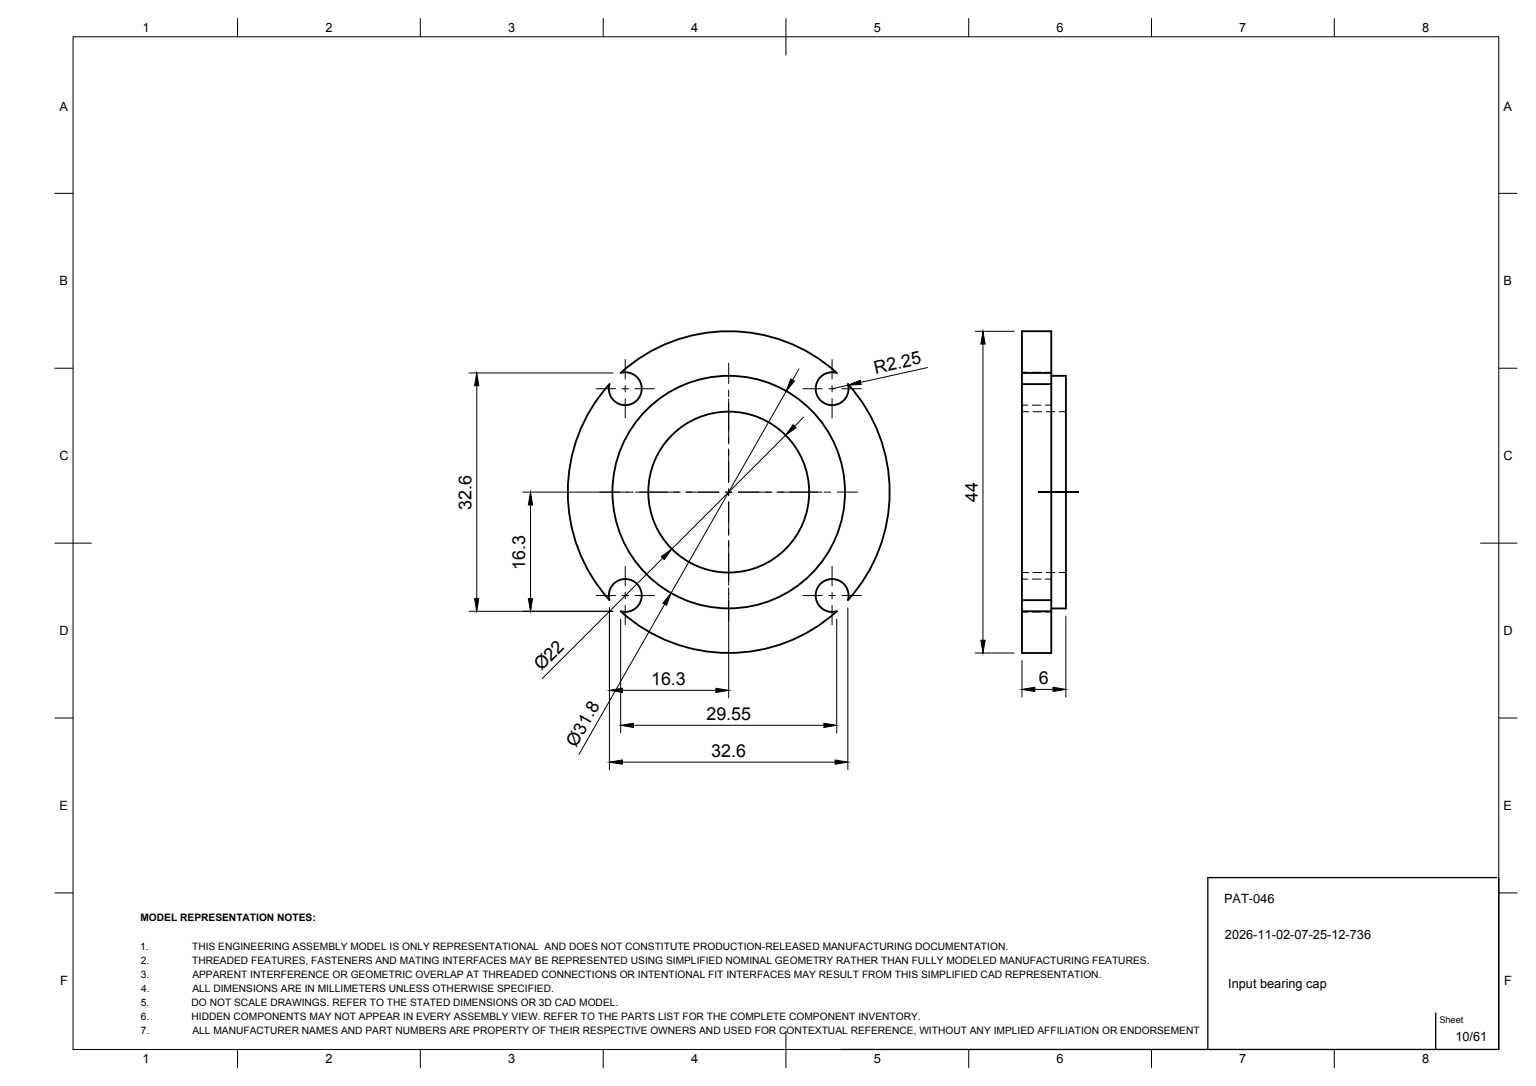
ISO-10303-21;
HEADER;
/* Generated by software containing ST-Developer
 * from STEP Tools, Inc. (www.steptools.com) 
 */

FILE_DESCRIPTION(
/* description */ ('Gear mesh backlash fixture'),
/* implementation_level */ '2;1');

FILE_NAME(
/* name */ 'Input bearing cap.step',
/* time_stamp */ '2026-10-28T03:26:00-07:00',
/* author */ (''),
/* organization */ (''),
/* preprocessor_version */ 'ST-DEVELOPER v20.2',
/* originating_system */ 'Autodesk Translation Framework v15.17.0.0',
/* authorisation */ '');

FILE_SCHEMA (('AUTOMOTIVE_DESIGN { 1 0 10303 214 3 1 1 }'));
ENDSEC;

DATA;
#10=MECHANICAL_DESIGN_GEOMETRIC_PRESENTATION_REPRESENTATION('',(#1021),#57900);
#921=SHAPE_REPRESENTATION_RELATIONSHIP('SRR','None',#58116,#971);
#971=ADVANCED_BREP_SHAPE_REPRESENTATION('',(#1086),#57849);
#1021=STYLED_ITEM('',(#58465),#1086);
#1086=MANIFOLD_SOLID_BREP('Body1',#13581);
#1187=FACE_BOUND('',#2571,.T.);
#1188=FACE_BOUND('',#2578,.T.);
#1189=FACE_BOUND('',#2581,.T.);
#1362=PLANE('',#14346);
#1363=PLANE('',#14362);
#1364=PLANE('',#14366);
#1757=FACE_OUTER_BOUND('',#2566,.T.);
#1758=FACE_OUTER_BOUND('',#2567,.T.);
#1759=FACE_OUTER_BOUND('',#2568,.T.);
#1760=FACE_OUTER_BOUND('',#2569,.T.);
#1761=FACE_OUTER_BOUND('',#2570,.T.);
#1762=FACE_OUTER_BOUND('',#2572,.T.);
#1763=FACE_OUTER_BOUND('',#2573,.T.);
#1764=FACE_OUTER_BOUND('',#2574,.T.);
#1765=FACE_OUTER_BOUND('',#2575,.T.);
#1766=FACE_OUTER_BOUND('',#2576,.T.);
#1767=FACE_OUTER_BOUND('',#2577,.T.);
#1768=FACE_OUTER_BOUND('',#2579,.T.);
#1769=FACE_OUTER_BOUND('',#2580,.T.);
#2566=EDGE_LOOP('',(#9165,#9166,#9167,#9168));
#2567=EDGE_LOOP('',(#9169,#9170,#9171,#9172));
#2568=EDGE_LOOP('',(#9173,#9174,#9175,#9176));
#2569=EDGE_LOOP('',(#9177,#9178,#9179,#9180));
#2570=EDGE_LOOP('',(#9181,#9182,#9183,#9184,#9185,#9186,#9187,#9188));
#2571=EDGE_LOOP('',(#9189));
#2572=EDGE_LOOP('',(#9190,#9191,#9192,#9193));
#2573=EDGE_LOOP('',(#9194,#9195,#9196,#9197));
#2574=EDGE_LOOP('',(#9198,#9199,#9200,#9201));
#2575=EDGE_LOOP('',(#9202,#9203,#9204,#9205));
#2576=EDGE_LOOP('',(#9206,#9207,#9208,#9209));
#2577=EDGE_LOOP('',(#9210));
#2578=EDGE_LOOP('',(#9211));
#2579=EDGE_LOOP('',(#9212,#9213,#9214,#9215));
#2580=EDGE_LOOP('',(#9216,#9217,#9218,#9219,#9220,#9221,#9222,#9223));
#2581=EDGE_LOOP('',(#9224));
#3482=LINE('',#19614,#4371);
#3483=LINE('',#19618,#4372);
#3484=LINE('',#19623,#4373);
#3485=LINE('',#19627,#4374);
#3486=LINE('',#19632,#4375);
#3487=LINE('',#19636,#4376);
#3488=LINE('',#19641,#4377);
#3489=LINE('',#19645,#4378);
#3490=LINE('',#19664,#4379);
#3491=LINE('',#19672,#4380);
#4371=VECTOR('',#15929,1.);
#4372=VECTOR('',#15932,1.);
#4373=VECTOR('',#15937,1.);
#4374=VECTOR('',#15940,1.);
#4375=VECTOR('',#15945,1.);
#4376=VECTOR('',#15948,1.);
#4377=VECTOR('',#15953,1.);
#4378=VECTOR('',#15956,1.);
#4379=VECTOR('',#15989,1.59);
#4380=VECTOR('',#16000,1.1);
#5257=CIRCLE('',#14335,0.225);
#5258=CIRCLE('',#14336,0.225);
#5259=CIRCLE('',#14338,0.225);
#5260=CIRCLE('',#14339,0.225);
#5261=CIRCLE('',#14341,0.225);
#5262=CIRCLE('',#14342,0.225);
#5263=CIRCLE('',#14344,0.225);
#5264=CIRCLE('',#14345,0.225);
#5265=CIRCLE('',#14347,2.2);
#5266=CIRCLE('',#14348,2.2);
#5267=CIRCLE('',#14349,2.2);
#5268=CIRCLE('',#14350,2.2);
#5269=CIRCLE('',#14351,1.59);
#5270=CIRCLE('',#14353,2.2);
#5271=CIRCLE('',#14355,2.2);
#5272=CIRCLE('',#14357,2.2);
#5273=CIRCLE('',#14359,2.2);
#5274=CIRCLE('',#14361,1.59);
#5275=CIRCLE('',#14363,1.1);
#5276=CIRCLE('',#14365,1.1);
#5877=VERTEX_POINT('',#19612);
#5878=VERTEX_POINT('',#19613);
#5879=VERTEX_POINT('',#19615);
#5880=VERTEX_POINT('',#19617);
#5881=VERTEX_POINT('',#19621);
#5882=VERTEX_POINT('',#19622);
#5883=VERTEX_POINT('',#19624);
#5884=VERTEX_POINT('',#19626);
#5885=VERTEX_POINT('',#19630);
#5886=VERTEX_POINT('',#19631);
#5887=VERTEX_POINT('',#19633);
#5888=VERTEX_POINT('',#19635);
#5889=VERTEX_POINT('',#19639);
#5890=VERTEX_POINT('',#19640);
#5891=VERTEX_POINT('',#19642);
#5892=VERTEX_POINT('',#19644);
#5893=VERTEX_POINT('',#19652);
#5894=VERTEX_POINT('',#19663);
#5895=VERTEX_POINT('',#19667);
#5896=VERTEX_POINT('',#19670);
#7169=EDGE_CURVE('',#5877,#5878,#3482,.T.);
#7170=EDGE_CURVE('',#5879,#5877,#5257,.T.);
#7171=EDGE_CURVE('',#5880,#5879,#3483,.T.);
#7172=EDGE_CURVE('',#5878,#5880,#5258,.T.);
#7173=EDGE_CURVE('',#5881,#5882,#3484,.T.);
#7174=EDGE_CURVE('',#5883,#5881,#5259,.T.);
#7175=EDGE_CURVE('',#5884,#5883,#3485,.T.);
#7176=EDGE_CURVE('',#5882,#5884,#5260,.T.);
#7177=EDGE_CURVE('',#5885,#5886,#3486,.T.);
#7178=EDGE_CURVE('',#5887,#5885,#5261,.T.);
#7179=EDGE_CURVE('',#5888,#5887,#3487,.T.);
#7180=EDGE_CURVE('',#5886,#5888,#5262,.T.);
#7181=EDGE_CURVE('',#5889,#5890,#3488,.T.);
#7182=EDGE_CURVE('',#5891,#5889,#5263,.T.);
#7183=EDGE_CURVE('',#5892,#5891,#3489,.T.);
#7184=EDGE_CURVE('',#5890,#5892,#5264,.T.);
#7185=EDGE_CURVE('',#5883,#5877,#5265,.T.);
#7186=EDGE_CURVE('',#5887,#5881,#5266,.T.);
#7187=EDGE_CURVE('',#5891,#5885,#5267,.T.);
#7188=EDGE_CURVE('',#5879,#5889,#5268,.T.);
#7189=EDGE_CURVE('',#5893,#5893,#5269,.T.);
#7190=EDGE_CURVE('',#5892,#5886,#5270,.T.);
#7191=EDGE_CURVE('',#5888,#5882,#5271,.T.);
#7192=EDGE_CURVE('',#5884,#5878,#5272,.T.);
#7193=EDGE_CURVE('',#5880,#5890,#5273,.T.);
#7194=EDGE_CURVE('',#5893,#5894,#3490,.T.);
#7195=EDGE_CURVE('',#5894,#5894,#5274,.T.);
#7196=EDGE_CURVE('',#5895,#5895,#5275,.T.);
#7197=EDGE_CURVE('',#5896,#5896,#5276,.T.);
#7198=EDGE_CURVE('',#5896,#5895,#3491,.T.);
#9165=ORIENTED_EDGE('',*,*,#7169,.F.);
#9166=ORIENTED_EDGE('',*,*,#7170,.F.);
#9167=ORIENTED_EDGE('',*,*,#7171,.F.);
#9168=ORIENTED_EDGE('',*,*,#7172,.F.);
#9169=ORIENTED_EDGE('',*,*,#7173,.F.);
#9170=ORIENTED_EDGE('',*,*,#7174,.F.);
#9171=ORIENTED_EDGE('',*,*,#7175,.F.);
#9172=ORIENTED_EDGE('',*,*,#7176,.F.);
#9173=ORIENTED_EDGE('',*,*,#7177,.F.);
#9174=ORIENTED_EDGE('',*,*,#7178,.F.);
#9175=ORIENTED_EDGE('',*,*,#7179,.F.);
#9176=ORIENTED_EDGE('',*,*,#7180,.F.);
#9177=ORIENTED_EDGE('',*,*,#7181,.F.);
#9178=ORIENTED_EDGE('',*,*,#7182,.F.);
#9179=ORIENTED_EDGE('',*,*,#7183,.F.);
#9180=ORIENTED_EDGE('',*,*,#7184,.F.);
#9181=ORIENTED_EDGE('',*,*,#7170,.T.);
#9182=ORIENTED_EDGE('',*,*,#7185,.F.);
#9183=ORIENTED_EDGE('',*,*,#7174,.T.);
#9184=ORIENTED_EDGE('',*,*,#7186,.F.);
#9185=ORIENTED_EDGE('',*,*,#7178,.T.);
#9186=ORIENTED_EDGE('',*,*,#7187,.F.);
#9187=ORIENTED_EDGE('',*,*,#7182,.T.);
#9188=ORIENTED_EDGE('',*,*,#7188,.F.);
#9189=ORIENTED_EDGE('',*,*,#7189,.T.);
#9190=ORIENTED_EDGE('',*,*,#7177,.T.);
#9191=ORIENTED_EDGE('',*,*,#7190,.F.);
#9192=ORIENTED_EDGE('',*,*,#7183,.T.);
#9193=ORIENTED_EDGE('',*,*,#7187,.T.);
#9194=ORIENTED_EDGE('',*,*,#7173,.T.);
#9195=ORIENTED_EDGE('',*,*,#7191,.F.);
#9196=ORIENTED_EDGE('',*,*,#7179,.T.);
#9197=ORIENTED_EDGE('',*,*,#7186,.T.);
#9198=ORIENTED_EDGE('',*,*,#7169,.T.);
#9199=ORIENTED_EDGE('',*,*,#7192,.F.);
#9200=ORIENTED_EDGE('',*,*,#7175,.T.);
#9201=ORIENTED_EDGE('',*,*,#7185,.T.);
#9202=ORIENTED_EDGE('',*,*,#7171,.T.);
#9203=ORIENTED_EDGE('',*,*,#7188,.T.);
#9204=ORIENTED_EDGE('',*,*,#7181,.T.);
#9205=ORIENTED_EDGE('',*,*,#7193,.F.);
#9206=ORIENTED_EDGE('',*,*,#7189,.F.);
#9207=ORIENTED_EDGE('',*,*,#7194,.T.);
#9208=ORIENTED_EDGE('',*,*,#7195,.T.);
#9209=ORIENTED_EDGE('',*,*,#7194,.F.);
#9210=ORIENTED_EDGE('',*,*,#7195,.F.);
#9211=ORIENTED_EDGE('',*,*,#7196,.F.);
#9212=ORIENTED_EDGE('',*,*,#7197,.F.);
#9213=ORIENTED_EDGE('',*,*,#7198,.T.);
#9214=ORIENTED_EDGE('',*,*,#7196,.T.);
#9215=ORIENTED_EDGE('',*,*,#7198,.F.);
#9216=ORIENTED_EDGE('',*,*,#7172,.T.);
#9217=ORIENTED_EDGE('',*,*,#7193,.T.);
#9218=ORIENTED_EDGE('',*,*,#7184,.T.);
#9219=ORIENTED_EDGE('',*,*,#7190,.T.);
#9220=ORIENTED_EDGE('',*,*,#7180,.T.);
#9221=ORIENTED_EDGE('',*,*,#7191,.T.);
#9222=ORIENTED_EDGE('',*,*,#7176,.T.);
#9223=ORIENTED_EDGE('',*,*,#7192,.T.);
#9224=ORIENTED_EDGE('',*,*,#7197,.T.);
#12616=CYLINDRICAL_SURFACE('',#14334,0.225);
#12617=CYLINDRICAL_SURFACE('',#14337,0.225);
#12618=CYLINDRICAL_SURFACE('',#14340,0.225);
#12619=CYLINDRICAL_SURFACE('',#14343,0.225);
#12620=CYLINDRICAL_SURFACE('',#14352,2.2);
#12621=CYLINDRICAL_SURFACE('',#14354,2.2);
#12622=CYLINDRICAL_SURFACE('',#14356,2.2);
#12623=CYLINDRICAL_SURFACE('',#14358,2.2);
#12624=CYLINDRICAL_SURFACE('',#14360,1.59);
#12625=CYLINDRICAL_SURFACE('',#14364,1.1);
#12874=ADVANCED_FACE('',(#1757),#12616,.F.);
#12875=ADVANCED_FACE('',(#1758),#12617,.F.);
#12876=ADVANCED_FACE('',(#1759),#12618,.F.);
#12877=ADVANCED_FACE('',(#1760),#12619,.F.);
#12878=ADVANCED_FACE('',(#1761,#1187),#1362,.F.);
#12879=ADVANCED_FACE('',(#1762),#12620,.T.);
#12880=ADVANCED_FACE('',(#1763),#12621,.T.);
#12881=ADVANCED_FACE('',(#1764),#12622,.T.);
#12882=ADVANCED_FACE('',(#1765),#12623,.T.);
#12883=ADVANCED_FACE('',(#1766),#12624,.T.);
#12884=ADVANCED_FACE('',(#1767,#1188),#1363,.F.);
#12885=ADVANCED_FACE('',(#1768),#12625,.F.);
#12886=ADVANCED_FACE('',(#1769,#1189),#1364,.T.);
#13581=CLOSED_SHELL('',(#12874,#12875,#12876,#12877,#12878,#12879,#12880,
#12881,#12882,#12883,#12884,#12885,#12886));
#14333=AXIS2_PLACEMENT_3D('',#19610,#15925,#15926);
#14334=AXIS2_PLACEMENT_3D('',#19611,#15927,#15928);
#14335=AXIS2_PLACEMENT_3D('',#19616,#15930,#15931);
#14336=AXIS2_PLACEMENT_3D('',#19619,#15933,#15934);
#14337=AXIS2_PLACEMENT_3D('',#19620,#15935,#15936);
#14338=AXIS2_PLACEMENT_3D('',#19625,#15938,#15939);
#14339=AXIS2_PLACEMENT_3D('',#19628,#15941,#15942);
#14340=AXIS2_PLACEMENT_3D('',#19629,#15943,#15944);
#14341=AXIS2_PLACEMENT_3D('',#19634,#15946,#15947);
#14342=AXIS2_PLACEMENT_3D('',#19637,#15949,#15950);
#14343=AXIS2_PLACEMENT_3D('',#19638,#15951,#15952);
#14344=AXIS2_PLACEMENT_3D('',#19643,#15954,#15955);
#14345=AXIS2_PLACEMENT_3D('',#19646,#15957,#15958);
#14346=AXIS2_PLACEMENT_3D('',#19647,#15959,#15960);
#14347=AXIS2_PLACEMENT_3D('',#19648,#15961,#15962);
#14348=AXIS2_PLACEMENT_3D('',#19649,#15963,#15964);
#14349=AXIS2_PLACEMENT_3D('',#19650,#15965,#15966);
#14350=AXIS2_PLACEMENT_3D('',#19651,#15967,#15968);
#14351=AXIS2_PLACEMENT_3D('',#19653,#15969,#15970);
#14352=AXIS2_PLACEMENT_3D('',#19654,#15971,#15972);
#14353=AXIS2_PLACEMENT_3D('',#19655,#15973,#15974);
#14354=AXIS2_PLACEMENT_3D('',#19656,#15975,#15976);
#14355=AXIS2_PLACEMENT_3D('',#19657,#15977,#15978);
#14356=AXIS2_PLACEMENT_3D('',#19658,#15979,#15980);
#14357=AXIS2_PLACEMENT_3D('',#19659,#15981,#15982);
#14358=AXIS2_PLACEMENT_3D('',#19660,#15983,#15984);
#14359=AXIS2_PLACEMENT_3D('',#19661,#15985,#15986);
#14360=AXIS2_PLACEMENT_3D('',#19662,#15987,#15988);
#14361=AXIS2_PLACEMENT_3D('',#19665,#15990,#15991);
#14362=AXIS2_PLACEMENT_3D('',#19666,#15992,#15993);
#14363=AXIS2_PLACEMENT_3D('',#19668,#15994,#15995);
#14364=AXIS2_PLACEMENT_3D('',#19669,#15996,#15997);
#14365=AXIS2_PLACEMENT_3D('',#19671,#15998,#15999);
#14366=AXIS2_PLACEMENT_3D('',#19673,#16001,#16002);
#15925=DIRECTION('axis',(0.,0.,1.));
#15926=DIRECTION('refdir',(1.,0.,0.));
#15927=DIRECTION('center_axis',(0.,0.,1.));
#15928=DIRECTION('ref_axis',(0.707106781186547,0.707106781186548,0.));
#15929=DIRECTION('',(0.,0.,1.));
#15930=DIRECTION('center_axis',(0.,0.,1.));
#15931=DIRECTION('ref_axis',(1.,0.,0.));
#15932=DIRECTION('',(0.,0.,-1.));
#15933=DIRECTION('center_axis',(0.,0.,-1.));
#15934=DIRECTION('ref_axis',(1.,0.,0.));
#15935=DIRECTION('center_axis',(0.,0.,1.));
#15936=DIRECTION('ref_axis',(0.707106781186548,-0.707106781186547,0.));
#15937=DIRECTION('',(0.,0.,1.));
#15938=DIRECTION('center_axis',(0.,0.,1.));
#15939=DIRECTION('ref_axis',(1.,0.,0.));
#15940=DIRECTION('',(0.,0.,-1.));
#15941=DIRECTION('center_axis',(0.,0.,-1.));
#15942=DIRECTION('ref_axis',(1.,0.,0.));
#15943=DIRECTION('center_axis',(0.,0.,1.));
#15944=DIRECTION('ref_axis',(-0.707106781186547,-0.707106781186548,0.));
#15945=DIRECTION('',(0.,0.,1.));
#15946=DIRECTION('center_axis',(0.,0.,1.));
#15947=DIRECTION('ref_axis',(1.,0.,0.));
#15948=DIRECTION('',(0.,0.,-1.));
#15949=DIRECTION('center_axis',(0.,0.,-1.));
#15950=DIRECTION('ref_axis',(1.,0.,0.));
#15951=DIRECTION('center_axis',(0.,0.,1.));
#15952=DIRECTION('ref_axis',(-0.707106781186548,0.707106781186547,0.));
#15953=DIRECTION('',(0.,0.,1.));
#15954=DIRECTION('center_axis',(0.,0.,1.));
#15955=DIRECTION('ref_axis',(1.,0.,0.));
#15956=DIRECTION('',(0.,0.,-1.));
#15957=DIRECTION('center_axis',(0.,0.,-1.));
#15958=DIRECTION('ref_axis',(1.,0.,0.));
#15959=DIRECTION('center_axis',(0.,0.,1.));
#15960=DIRECTION('ref_axis',(1.,0.,0.));
#15961=DIRECTION('center_axis',(0.,0.,1.));
#15962=DIRECTION('ref_axis',(1.,0.,0.));
#15963=DIRECTION('center_axis',(0.,0.,1.));
#15964=DIRECTION('ref_axis',(1.,0.,0.));
#15965=DIRECTION('center_axis',(0.,0.,1.));
#15966=DIRECTION('ref_axis',(1.,0.,0.));
#15967=DIRECTION('center_axis',(0.,0.,1.));
#15968=DIRECTION('ref_axis',(1.,0.,0.));
#15969=DIRECTION('center_axis',(0.,0.,1.));
#15970=DIRECTION('ref_axis',(1.,0.,0.));
#15971=DIRECTION('center_axis',(0.,0.,1.));
#15972=DIRECTION('ref_axis',(1.,0.,0.));
#15973=DIRECTION('center_axis',(0.,0.,1.));
#15974=DIRECTION('ref_axis',(1.,0.,0.));
#15975=DIRECTION('center_axis',(0.,0.,1.));
#15976=DIRECTION('ref_axis',(1.,0.,0.));
#15977=DIRECTION('center_axis',(0.,0.,1.));
#15978=DIRECTION('ref_axis',(1.,0.,0.));
#15979=DIRECTION('center_axis',(0.,0.,1.));
#15980=DIRECTION('ref_axis',(-1.,-1.22464679914735E-16,0.));
#15981=DIRECTION('center_axis',(0.,0.,1.));
#15982=DIRECTION('ref_axis',(1.,0.,0.));
#15983=DIRECTION('center_axis',(0.,0.,1.));
#15984=DIRECTION('ref_axis',(1.,0.,0.));
#15985=DIRECTION('center_axis',(0.,0.,1.));
#15986=DIRECTION('ref_axis',(1.,0.,0.));
#15987=DIRECTION('center_axis',(0.,0.,1.));
#15988=DIRECTION('ref_axis',(1.,0.,0.));
#15989=DIRECTION('',(0.,0.,-1.));
#15990=DIRECTION('center_axis',(0.,0.,1.));
#15991=DIRECTION('ref_axis',(1.,0.,0.));
#15992=DIRECTION('center_axis',(0.,0.,1.));
#15993=DIRECTION('ref_axis',(1.,0.,0.));
#15994=DIRECTION('center_axis',(0.,0.,-1.));
#15995=DIRECTION('ref_axis',(1.,0.,0.));
#15996=DIRECTION('center_axis',(0.,0.,1.));
#15997=DIRECTION('ref_axis',(1.,0.,0.));
#15998=DIRECTION('center_axis',(0.,0.,-1.));
#15999=DIRECTION('ref_axis',(1.,0.,0.));
#16000=DIRECTION('',(0.,0.,-1.));
#16001=DIRECTION('center_axis',(0.,0.,1.));
#16002=DIRECTION('ref_axis',(1.,0.,0.));
#19610=CARTESIAN_POINT('',(0.,0.,0.));
#19611=CARTESIAN_POINT('Origin',(-1.4142135623731,-1.41421356237309,9.1));
#19612=CARTESIAN_POINT('',(-1.6301780125076,-1.47733531993816,9.2));
#19613=CARTESIAN_POINT('',(-1.6301780125076,-1.47733531993816,9.6));
#19614=CARTESIAN_POINT('',(-1.6301780125076,-1.47733531993816,9.1));
#19615=CARTESIAN_POINT('',(-1.47733531993816,-1.6301780125076,9.2));
#19616=CARTESIAN_POINT('Origin',(-1.4142135623731,-1.41421356237309,9.2));
#19617=CARTESIAN_POINT('',(-1.47733531993816,-1.6301780125076,9.6));
#19618=CARTESIAN_POINT('',(-1.47733531993816,-1.6301780125076,9.1));
#19619=CARTESIAN_POINT('Origin',(-1.4142135623731,-1.41421356237309,9.6));
#19620=CARTESIAN_POINT('Origin',(-1.41421356237309,1.4142135623731,9.1));
#19621=CARTESIAN_POINT('',(-1.47733531993816,1.6301780125076,9.2));
#19622=CARTESIAN_POINT('',(-1.47733531993816,1.6301780125076,9.6));
#19623=CARTESIAN_POINT('',(-1.47733531993816,1.6301780125076,9.1));
#19624=CARTESIAN_POINT('',(-1.6301780125076,1.47733531993816,9.2));
#19625=CARTESIAN_POINT('Origin',(-1.41421356237309,1.4142135623731,9.2));
#19626=CARTESIAN_POINT('',(-1.6301780125076,1.47733531993816,9.6));
#19627=CARTESIAN_POINT('',(-1.6301780125076,1.47733531993816,9.1));
#19628=CARTESIAN_POINT('Origin',(-1.41421356237309,1.4142135623731,9.6));
#19629=CARTESIAN_POINT('Origin',(1.4142135623731,1.41421356237309,9.1));
#19630=CARTESIAN_POINT('',(1.6301780125076,1.47733531993816,9.2));
#19631=CARTESIAN_POINT('',(1.6301780125076,1.47733531993816,9.6));
#19632=CARTESIAN_POINT('',(1.6301780125076,1.47733531993816,9.1));
#19633=CARTESIAN_POINT('',(1.47733531993816,1.6301780125076,9.2));
#19634=CARTESIAN_POINT('Origin',(1.4142135623731,1.41421356237309,9.2));
#19635=CARTESIAN_POINT('',(1.47733531993816,1.6301780125076,9.6));
#19636=CARTESIAN_POINT('',(1.47733531993816,1.6301780125076,9.1));
#19637=CARTESIAN_POINT('Origin',(1.4142135623731,1.41421356237309,9.6));
#19638=CARTESIAN_POINT('Origin',(1.41421356237309,-1.4142135623731,9.1));
#19639=CARTESIAN_POINT('',(1.47733531993816,-1.6301780125076,9.2));
#19640=CARTESIAN_POINT('',(1.47733531993816,-1.6301780125076,9.6));
#19641=CARTESIAN_POINT('',(1.47733531993816,-1.6301780125076,9.1));
#19642=CARTESIAN_POINT('',(1.6301780125076,-1.47733531993816,9.2));
#19643=CARTESIAN_POINT('Origin',(1.41421356237309,-1.4142135623731,9.2));
#19644=CARTESIAN_POINT('',(1.6301780125076,-1.47733531993816,9.6));
#19645=CARTESIAN_POINT('',(1.6301780125076,-1.47733531993816,9.1));
#19646=CARTESIAN_POINT('Origin',(1.41421356237309,-1.4142135623731,9.6));
#19647=CARTESIAN_POINT('Origin',(0.,0.,9.2));
#19648=CARTESIAN_POINT('Origin',(0.,0.,9.2));
#19649=CARTESIAN_POINT('Origin',(0.,0.,9.2));
#19650=CARTESIAN_POINT('Origin',(0.,0.,9.2));
#19651=CARTESIAN_POINT('Origin',(0.,0.,9.2));
#19652=CARTESIAN_POINT('',(-1.59,-1.94718841064429E-16,9.2));
#19653=CARTESIAN_POINT('Origin',(0.,0.,9.2));
#19654=CARTESIAN_POINT('Origin',(0.,0.,9.2));
#19655=CARTESIAN_POINT('Origin',(0.,0.,9.6));
#19656=CARTESIAN_POINT('Origin',(0.,0.,9.2));
#19657=CARTESIAN_POINT('Origin',(0.,0.,9.6));
#19658=CARTESIAN_POINT('Origin',(0.,0.,9.2));
#19659=CARTESIAN_POINT('Origin',(0.,0.,9.6));
#19660=CARTESIAN_POINT('Origin',(0.,0.,9.2));
#19661=CARTESIAN_POINT('Origin',(0.,0.,9.6));
#19662=CARTESIAN_POINT('Origin',(0.,0.,9.));
#19663=CARTESIAN_POINT('',(-1.59,-1.94718841064429E-16,9.));
#19664=CARTESIAN_POINT('',(-1.59,-1.94718841064429E-16,9.));
#19665=CARTESIAN_POINT('Origin',(0.,0.,9.));
#19666=CARTESIAN_POINT('Origin',(0.,0.,9.));
#19667=CARTESIAN_POINT('',(-1.1,-1.34711147906209E-16,9.));
#19668=CARTESIAN_POINT('Origin',(0.,0.,9.));
#19669=CARTESIAN_POINT('Origin',(0.,0.,9.2));
#19670=CARTESIAN_POINT('',(-1.1,-1.34711147906209E-16,9.6));
#19671=CARTESIAN_POINT('Origin',(0.,0.,9.6));
#19672=CARTESIAN_POINT('',(-1.1,-1.34711147906209E-16,9.2));
#19673=CARTESIAN_POINT('Origin',(0.,0.,9.6));
#57790=UNCERTAINTY_MEASURE_WITH_UNIT(LENGTH_MEASURE(0.001),#57901,
'DISTANCE_ACCURACY_VALUE',
'Maximum model space distance between geometric entities at asserted c
onnectivities');
#57841=UNCERTAINTY_MEASURE_WITH_UNIT(LENGTH_MEASURE(0.001),#57901,
'DISTANCE_ACCURACY_VALUE',
'Maximum model space distance between geometric entities at asserted c
onnectivities');
#57849=(
GEOMETRIC_REPRESENTATION_CONTEXT(3)
GLOBAL_UNCERTAINTY_ASSIGNED_CONTEXT((#57790))
GLOBAL_UNIT_ASSIGNED_CONTEXT((#57901,#57903,#57904))
REPRESENTATION_CONTEXT('','3D')
);
#57900=(
GEOMETRIC_REPRESENTATION_CONTEXT(3)
GLOBAL_UNCERTAINTY_ASSIGNED_CONTEXT((#57841))
GLOBAL_UNIT_ASSIGNED_CONTEXT((#57901,#57903,#57904))
REPRESENTATION_CONTEXT('','3D')
);
#57901=(
LENGTH_UNIT()
NAMED_UNIT(*)
SI_UNIT(.CENTI.,.METRE.)
);
#57903=(
NAMED_UNIT(*)
PLANE_ANGLE_UNIT()
SI_UNIT($,.RADIAN.)
);
#57904=(
NAMED_UNIT(*)
SI_UNIT($,.STERADIAN.)
SOLID_ANGLE_UNIT()
);
#57912=SHAPE_DEFINITION_REPRESENTATION(#57970,#58116);
#57970=PRODUCT_DEFINITION_SHAPE('',$,#58175);
#58116=SHAPE_REPRESENTATION('',(#14333),#57849);
#58167=PRODUCT_DEFINITION_CONTEXT('part definition',#58343,'design');
#58175=PRODUCT_DEFINITION('Input bearing cap','Input bearing cap',#58233,
#58167);
#58233=PRODUCT_DEFINITION_FORMATION('',$,#58352);
#58343=APPLICATION_CONTEXT(
'Core Data for Automotive Mechanical Design Process');
#58344=PRODUCT_CONTEXT('part definition',#58343,'mechanical');
#58352=PRODUCT('Input bearing cap','Input bearing cap',
'Input bearing cap',(#58344));
#58459=COLOUR_RGB('Grey',0.48,0.52,0.57);
#58460=FILL_AREA_STYLE_COLOUR('',#58459);
#58461=FILL_AREA_STYLE('',(#58460));
#58462=SURFACE_STYLE_FILL_AREA(#58461);
#58463=SURFACE_SIDE_STYLE('',(#58462));
#58464=SURFACE_STYLE_USAGE(.BOTH.,#58463);
#58465=PRESENTATION_STYLE_ASSIGNMENT((#58464));
ENDSEC;
END-ISO-10303-21;
